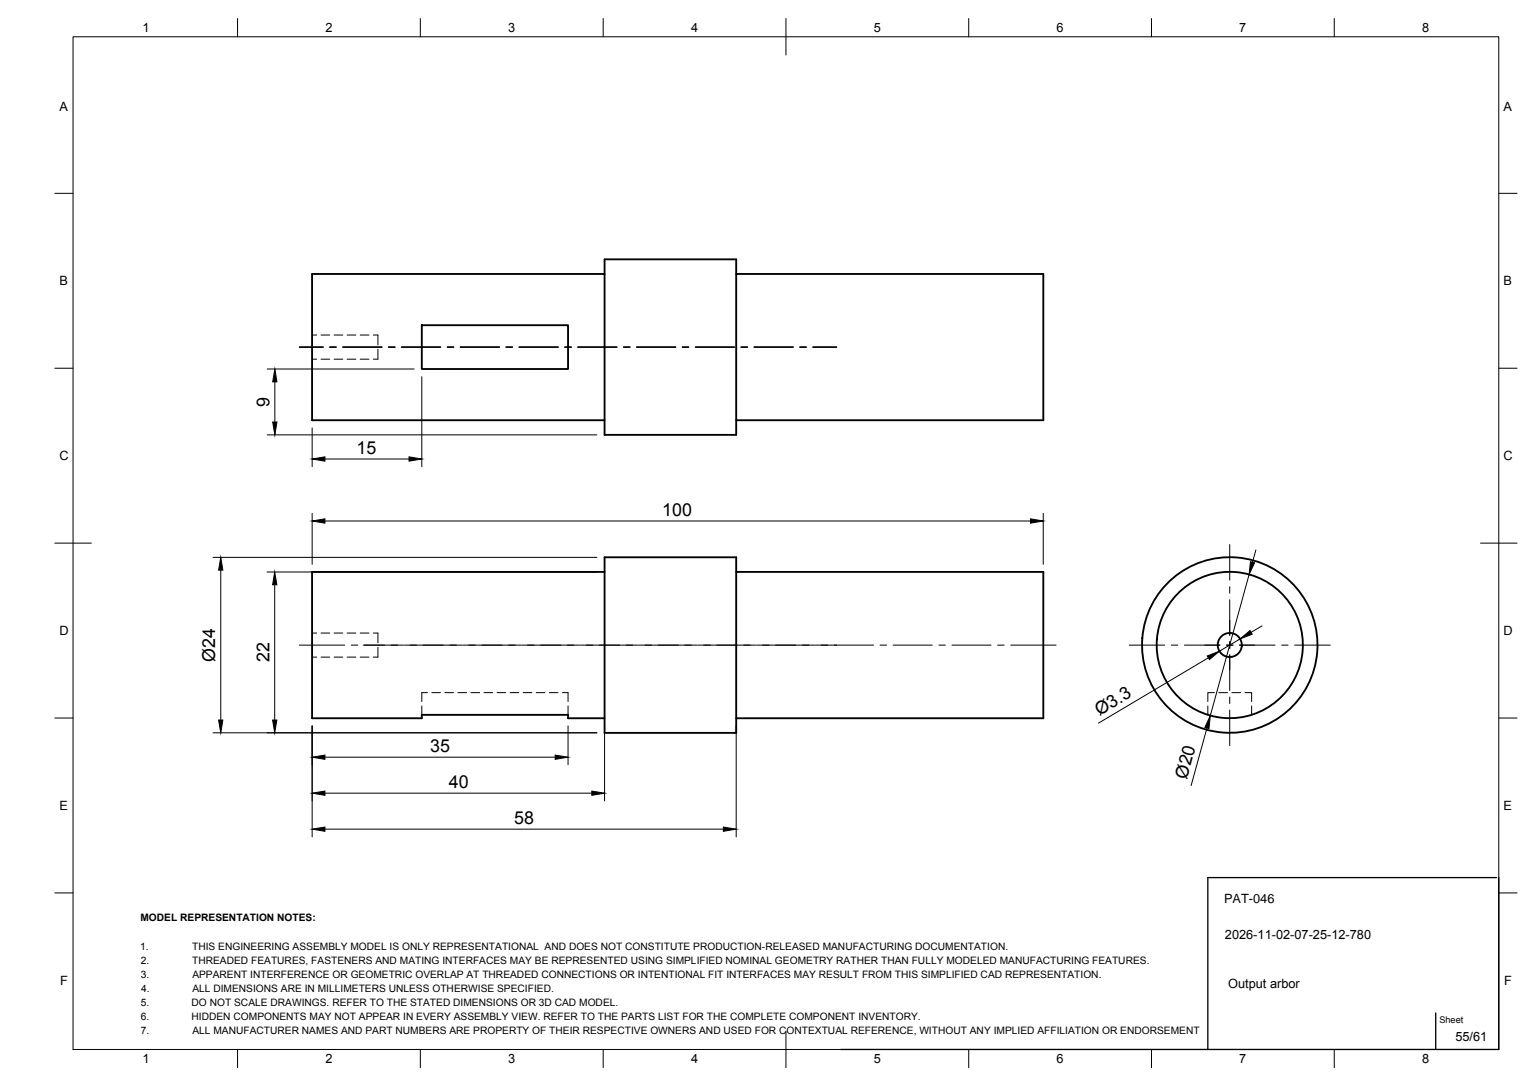
ISO-10303-21;
HEADER;
/* Generated by software containing ST-Developer
 * from STEP Tools, Inc. (www.steptools.com) 
 */

FILE_DESCRIPTION(
/* description */ ('Gear mesh backlash fixture'),
/* implementation_level */ '2;1');

FILE_NAME(
/* name */ 'Output arbor.step',
/* time_stamp */ '2026-10-28T03:26:00-07:00',
/* author */ (''),
/* organization */ (''),
/* preprocessor_version */ 'ST-DEVELOPER v20.2',
/* originating_system */ 'Autodesk Translation Framework v15.17.0.0',
/* authorisation */ '');

FILE_SCHEMA (('AUTOMOTIVE_DESIGN { 1 0 10303 214 3 1 1 }'));
ENDSEC;

DATA;
#10=MECHANICAL_DESIGN_GEOMETRIC_PRESENTATION_REPRESENTATION('',(#1072),#57900);
#957=SHAPE_REPRESENTATION_RELATIONSHIP('SRR','None',#58158,#1007);
#1007=ADVANCED_BREP_SHAPE_REPRESENTATION('',(#1135),#57891);
#1072=STYLED_ITEM('',(#58479),#1135);
#1135=MANIFOLD_SOLID_BREP('Body1',#13634);
#1311=FACE_BOUND('',#3168,.T.);
#1312=FACE_BOUND('',#3170,.T.);
#1313=FACE_BOUND('',#3174,.T.);
#1314=FACE_BOUND('',#3176,.T.);
#1604=PLANE('',#15226);
#1605=PLANE('',#15227);
#1606=PLANE('',#15228);
#1607=PLANE('',#15230);
#1608=PLANE('',#15231);
#1609=PLANE('',#15232);
#1610=PLANE('',#15234);
#1611=PLANE('',#15237);
#1612=PLANE('',#15245);
#1613=PLANE('',#15246);
#2227=FACE_OUTER_BOUND('',#3160,.T.);
#2228=FACE_OUTER_BOUND('',#3161,.T.);
#2229=FACE_OUTER_BOUND('',#3162,.T.);
#2230=FACE_OUTER_BOUND('',#3163,.T.);
#2231=FACE_OUTER_BOUND('',#3164,.T.);
#2232=FACE_OUTER_BOUND('',#3165,.T.);
#2233=FACE_OUTER_BOUND('',#3166,.T.);
#2234=FACE_OUTER_BOUND('',#3167,.T.);
#2235=FACE_OUTER_BOUND('',#3169,.T.);
#2236=FACE_OUTER_BOUND('',#3171,.T.);
#2237=FACE_OUTER_BOUND('',#3172,.T.);
#2238=FACE_OUTER_BOUND('',#3173,.T.);
#2239=FACE_OUTER_BOUND('',#3175,.T.);
#2240=FACE_OUTER_BOUND('',#3177,.T.);
#3160=EDGE_LOOP('',(#11359,#11360,#11361,#11362));
#3161=EDGE_LOOP('',(#11363));
#3162=EDGE_LOOP('',(#11364,#11365,#11366,#11367));
#3163=EDGE_LOOP('',(#11368,#11369,#11370,#11371));
#3164=EDGE_LOOP('',(#11372,#11373,#11374,#11375));
#3165=EDGE_LOOP('',(#11376,#11377,#11378,#11379));
#3166=EDGE_LOOP('',(#11380,#11381,#11382,#11383));
#3167=EDGE_LOOP('',(#11384));
#3168=EDGE_LOOP('',(#11385));
#3169=EDGE_LOOP('',(#11386));
#3170=EDGE_LOOP('',(#11387));
#3171=EDGE_LOOP('',(#11388,#11389,#11390,#11391));
#3172=EDGE_LOOP('',(#11392,#11393,#11394,#11395));
#3173=EDGE_LOOP('',(#11396,#11397,#11398,#11399));
#3174=EDGE_LOOP('',(#11400,#11401,#11402,#11403));
#3175=EDGE_LOOP('',(#11404));
#3176=EDGE_LOOP('',(#11405));
#3177=EDGE_LOOP('',(#11406));
#4051=LINE('',#33823,#4940);
#4052=LINE('',#33829,#4941);
#4053=LINE('',#33831,#4942);
#4054=LINE('',#33833,#4943);
#4055=LINE('',#33834,#4944);
#4056=LINE('',#33839,#4945);
#4057=LINE('',#33840,#4946);
#4058=LINE('',#33843,#4947);
#4059=LINE('',#33844,#4948);
#4060=LINE('',#33847,#4949);
#4061=LINE('',#33848,#4950);
#4062=LINE('',#33862,#4951);
#4063=LINE('',#33865,#4952);
#4064=LINE('',#33870,#4953);
#4940=VECTOR('',#18278,0.165);
#4941=VECTOR('',#18285,1.);
#4942=VECTOR('',#18286,1.);
#4943=VECTOR('',#18287,1.);
#4944=VECTOR('',#18288,1.);
#4945=VECTOR('',#18293,1.);
#4946=VECTOR('',#18294,1.);
#4947=VECTOR('',#18297,1.);
#4948=VECTOR('',#18298,1.);
#4949=VECTOR('',#18301,1.);
#4950=VECTOR('',#18302,1.);
#4951=VECTOR('',#18321,1.2);
#4952=VECTOR('',#18324,1.);
#4953=VECTOR('',#18331,1.);
#5661=CIRCLE('',#15224,0.165);
#5662=CIRCLE('',#15225,0.165);
#5663=CIRCLE('',#15229,1.);
#5664=CIRCLE('',#15233,1.);
#5665=CIRCLE('',#15235,1.2);
#5666=CIRCLE('',#15236,1.);
#5667=CIRCLE('',#15238,1.2);
#5668=CIRCLE('',#15239,1.);
#5669=CIRCLE('',#15242,1.);
#5670=CIRCLE('',#15244,1.);
#6618=VERTEX_POINT('',#33820);
#6619=VERTEX_POINT('',#33822);
#6620=VERTEX_POINT('',#33827);
#6621=VERTEX_POINT('',#33828);
#6622=VERTEX_POINT('',#33830);
#6623=VERTEX_POINT('',#33832);
#6624=VERTEX_POINT('',#33836);
#6625=VERTEX_POINT('',#33838);
#6626=VERTEX_POINT('',#33842);
#6627=VERTEX_POINT('',#33846);
#6628=VERTEX_POINT('',#33852);
#6629=VERTEX_POINT('',#33854);
#6630=VERTEX_POINT('',#33857);
#6631=VERTEX_POINT('',#33859);
#6632=VERTEX_POINT('',#33864);
#6633=VERTEX_POINT('',#33868);
#8266=EDGE_CURVE('',#6618,#6618,#5661,.T.);
#8267=EDGE_CURVE('',#6618,#6619,#4051,.T.);
#8268=EDGE_CURVE('',#6619,#6619,#5662,.T.);
#8269=EDGE_CURVE('',#6620,#6621,#4052,.T.);
#8270=EDGE_CURVE('',#6620,#6622,#4053,.T.);
#8271=EDGE_CURVE('',#6623,#6622,#4054,.T.);
#8272=EDGE_CURVE('',#6623,#6621,#4055,.T.);
#8273=EDGE_CURVE('',#6621,#6624,#5663,.T.);
#8274=EDGE_CURVE('',#6625,#6623,#4056,.T.);
#8275=EDGE_CURVE('',#6624,#6625,#4057,.T.);
#8276=EDGE_CURVE('',#6622,#6626,#4058,.T.);
#8277=EDGE_CURVE('',#6625,#6626,#4059,.T.);
#8278=EDGE_CURVE('',#6624,#6627,#4060,.T.);
#8279=EDGE_CURVE('',#6626,#6627,#4061,.T.);
#8280=EDGE_CURVE('',#6627,#6620,#5664,.T.);
#8281=EDGE_CURVE('',#6628,#6628,#5665,.T.);
#8282=EDGE_CURVE('',#6629,#6629,#5666,.T.);
#8283=EDGE_CURVE('',#6630,#6630,#5667,.T.);
#8284=EDGE_CURVE('',#6631,#6631,#5668,.T.);
#8285=EDGE_CURVE('',#6628,#6630,#4062,.T.);
#8286=EDGE_CURVE('',#6631,#6632,#4063,.T.);
#8287=EDGE_CURVE('',#6632,#6632,#5669,.T.);
#8288=EDGE_CURVE('',#6633,#6633,#5670,.T.);
#8289=EDGE_CURVE('',#6633,#6629,#4064,.T.);
#11359=ORIENTED_EDGE('',*,*,#8266,.F.);
#11360=ORIENTED_EDGE('',*,*,#8267,.T.);
#11361=ORIENTED_EDGE('',*,*,#8268,.F.);
#11362=ORIENTED_EDGE('',*,*,#8267,.F.);
#11363=ORIENTED_EDGE('',*,*,#8266,.T.);
#11364=ORIENTED_EDGE('',*,*,#8269,.F.);
#11365=ORIENTED_EDGE('',*,*,#8270,.T.);
#11366=ORIENTED_EDGE('',*,*,#8271,.F.);
#11367=ORIENTED_EDGE('',*,*,#8272,.T.);
#11368=ORIENTED_EDGE('',*,*,#8273,.F.);
#11369=ORIENTED_EDGE('',*,*,#8272,.F.);
#11370=ORIENTED_EDGE('',*,*,#8274,.F.);
#11371=ORIENTED_EDGE('',*,*,#8275,.F.);
#11372=ORIENTED_EDGE('',*,*,#8274,.T.);
#11373=ORIENTED_EDGE('',*,*,#8271,.T.);
#11374=ORIENTED_EDGE('',*,*,#8276,.T.);
#11375=ORIENTED_EDGE('',*,*,#8277,.F.);
#11376=ORIENTED_EDGE('',*,*,#8278,.F.);
#11377=ORIENTED_EDGE('',*,*,#8275,.T.);
#11378=ORIENTED_EDGE('',*,*,#8277,.T.);
#11379=ORIENTED_EDGE('',*,*,#8279,.T.);
#11380=ORIENTED_EDGE('',*,*,#8280,.F.);
#11381=ORIENTED_EDGE('',*,*,#8279,.F.);
#11382=ORIENTED_EDGE('',*,*,#8276,.F.);
#11383=ORIENTED_EDGE('',*,*,#8270,.F.);
#11384=ORIENTED_EDGE('',*,*,#8281,.T.);
#11385=ORIENTED_EDGE('',*,*,#8282,.F.);
#11386=ORIENTED_EDGE('',*,*,#8283,.F.);
#11387=ORIENTED_EDGE('',*,*,#8284,.F.);
#11388=ORIENTED_EDGE('',*,*,#8281,.F.);
#11389=ORIENTED_EDGE('',*,*,#8285,.T.);
#11390=ORIENTED_EDGE('',*,*,#8283,.T.);
#11391=ORIENTED_EDGE('',*,*,#8285,.F.);
#11392=ORIENTED_EDGE('',*,*,#8284,.T.);
#11393=ORIENTED_EDGE('',*,*,#8286,.T.);
#11394=ORIENTED_EDGE('',*,*,#8287,.T.);
#11395=ORIENTED_EDGE('',*,*,#8286,.F.);
#11396=ORIENTED_EDGE('',*,*,#8288,.F.);
#11397=ORIENTED_EDGE('',*,*,#8289,.T.);
#11398=ORIENTED_EDGE('',*,*,#8282,.T.);
#11399=ORIENTED_EDGE('',*,*,#8289,.F.);
#11400=ORIENTED_EDGE('',*,*,#8278,.T.);
#11401=ORIENTED_EDGE('',*,*,#8280,.T.);
#11402=ORIENTED_EDGE('',*,*,#8269,.T.);
#11403=ORIENTED_EDGE('',*,*,#8273,.T.);
#11404=ORIENTED_EDGE('',*,*,#8288,.T.);
#11405=ORIENTED_EDGE('',*,*,#8268,.T.);
#11406=ORIENTED_EDGE('',*,*,#8287,.F.);
#12753=CYLINDRICAL_SURFACE('',#15223,0.165);
#12754=CYLINDRICAL_SURFACE('',#15240,1.2);
#12755=CYLINDRICAL_SURFACE('',#15241,1.);
#12756=CYLINDRICAL_SURFACE('',#15243,1.);
#13344=ADVANCED_FACE('',(#2227),#12753,.F.);
#13345=ADVANCED_FACE('',(#2228),#1604,.T.);
#13346=ADVANCED_FACE('',(#2229),#1605,.F.);
#13347=ADVANCED_FACE('',(#2230),#1606,.T.);
#13348=ADVANCED_FACE('',(#2231),#1607,.F.);
#13349=ADVANCED_FACE('',(#2232),#1608,.F.);
#13350=ADVANCED_FACE('',(#2233),#1609,.F.);
#13351=ADVANCED_FACE('',(#2234,#1311),#1610,.T.);
#13352=ADVANCED_FACE('',(#2235,#1312),#1611,.F.);
#13353=ADVANCED_FACE('',(#2236),#12754,.T.);
#13354=ADVANCED_FACE('',(#2237),#12755,.T.);
#13355=ADVANCED_FACE('',(#2238,#1313),#12756,.T.);
#13356=ADVANCED_FACE('',(#2239,#1314),#1612,.T.);
#13357=ADVANCED_FACE('',(#2240),#1613,.F.);
#13634=CLOSED_SHELL('',(#13344,#13345,#13346,#13347,#13348,#13349,#13350,
#13351,#13352,#13353,#13354,#13355,#13356,#13357));
#15222=AXIS2_PLACEMENT_3D('',#33818,#18272,#18273);
#15223=AXIS2_PLACEMENT_3D('',#33819,#18274,#18275);
#15224=AXIS2_PLACEMENT_3D('',#33821,#18276,#18277);
#15225=AXIS2_PLACEMENT_3D('',#33824,#18279,#18280);
#15226=AXIS2_PLACEMENT_3D('',#33825,#18281,#18282);
#15227=AXIS2_PLACEMENT_3D('',#33826,#18283,#18284);
#15228=AXIS2_PLACEMENT_3D('',#33835,#18289,#18290);
#15229=AXIS2_PLACEMENT_3D('',#33837,#18291,#18292);
#15230=AXIS2_PLACEMENT_3D('',#33841,#18295,#18296);
#15231=AXIS2_PLACEMENT_3D('',#33845,#18299,#18300);
#15232=AXIS2_PLACEMENT_3D('',#33849,#18303,#18304);
#15233=AXIS2_PLACEMENT_3D('',#33850,#18305,#18306);
#15234=AXIS2_PLACEMENT_3D('',#33851,#18307,#18308);
#15235=AXIS2_PLACEMENT_3D('',#33853,#18309,#18310);
#15236=AXIS2_PLACEMENT_3D('',#33855,#18311,#18312);
#15237=AXIS2_PLACEMENT_3D('',#33856,#18313,#18314);
#15238=AXIS2_PLACEMENT_3D('',#33858,#18315,#18316);
#15239=AXIS2_PLACEMENT_3D('',#33860,#18317,#18318);
#15240=AXIS2_PLACEMENT_3D('',#33861,#18319,#18320);
#15241=AXIS2_PLACEMENT_3D('',#33863,#18322,#18323);
#15242=AXIS2_PLACEMENT_3D('',#33866,#18325,#18326);
#15243=AXIS2_PLACEMENT_3D('',#33867,#18327,#18328);
#15244=AXIS2_PLACEMENT_3D('',#33869,#18329,#18330);
#15245=AXIS2_PLACEMENT_3D('',#33871,#18332,#18333);
#15246=AXIS2_PLACEMENT_3D('',#33872,#18334,#18335);
#18272=DIRECTION('axis',(0.,0.,1.));
#18273=DIRECTION('refdir',(1.,0.,0.));
#18274=DIRECTION('center_axis',(0.,0.,1.));
#18275=DIRECTION('ref_axis',(1.,0.,0.));
#18276=DIRECTION('center_axis',(0.,0.,1.));
#18277=DIRECTION('ref_axis',(1.,0.,0.));
#18278=DIRECTION('',(0.,0.,1.));
#18279=DIRECTION('center_axis',(0.,0.,-1.));
#18280=DIRECTION('ref_axis',(1.,0.,0.));
#18281=DIRECTION('center_axis',(0.,0.,1.));
#18282=DIRECTION('ref_axis',(1.,0.,0.));
#18283=DIRECTION('center_axis',(-0.996917333733128,-0.0784590957278475,
0.));
#18284=DIRECTION('ref_axis',(0.0784590957278475,-0.996917333733128,0.));
#18285=DIRECTION('',(0.,0.,-1.));
#18286=DIRECTION('',(0.0784590957278475,-0.996917333733128,0.));
#18287=DIRECTION('',(0.,0.,1.));
#18288=DIRECTION('',(-0.0784590957278475,0.996917333733128,0.));
#18289=DIRECTION('center_axis',(0.,0.,1.));
#18290=DIRECTION('ref_axis',(1.,0.,0.));
#18291=DIRECTION('center_axis',(0.,0.,-1.));
#18292=DIRECTION('ref_axis',(1.,0.,0.));
#18293=DIRECTION('',(-0.996917333733128,-0.0784590957278448,0.));
#18294=DIRECTION('',(0.0784590957278475,-0.996917333733128,0.));
#18295=DIRECTION('center_axis',(0.0784590957278448,-0.996917333733128,0.));
#18296=DIRECTION('ref_axis',(0.996917333733128,0.0784590957278448,0.));
#18297=DIRECTION('',(0.996917333733128,0.0784590957278448,0.));
#18298=DIRECTION('',(0.,0.,1.));
#18299=DIRECTION('center_axis',(0.996917333733128,0.0784590957278475,0.));
#18300=DIRECTION('ref_axis',(-0.0784590957278475,0.996917333733128,0.));
#18301=DIRECTION('',(0.,0.,1.));
#18302=DIRECTION('',(-0.0784590957278475,0.996917333733128,0.));
#18303=DIRECTION('center_axis',(0.,0.,1.));
#18304=DIRECTION('ref_axis',(1.,0.,0.));
#18305=DIRECTION('center_axis',(0.,0.,1.));
#18306=DIRECTION('ref_axis',(1.,0.,0.));
#18307=DIRECTION('center_axis',(0.,0.,1.));
#18308=DIRECTION('ref_axis',(1.,0.,0.));
#18309=DIRECTION('center_axis',(0.,0.,1.));
#18310=DIRECTION('ref_axis',(1.,0.,0.));
#18311=DIRECTION('center_axis',(0.,0.,1.));
#18312=DIRECTION('ref_axis',(1.,0.,0.));
#18313=DIRECTION('center_axis',(0.,0.,1.));
#18314=DIRECTION('ref_axis',(1.,0.,0.));
#18315=DIRECTION('center_axis',(0.,0.,1.));
#18316=DIRECTION('ref_axis',(1.,0.,0.));
#18317=DIRECTION('center_axis',(0.,0.,-1.));
#18318=DIRECTION('ref_axis',(1.,0.,0.));
#18319=DIRECTION('center_axis',(0.,0.,1.));
#18320=DIRECTION('ref_axis',(1.,0.,0.));
#18321=DIRECTION('',(0.,0.,-1.));
#18322=DIRECTION('center_axis',(0.,0.,1.));
#18323=DIRECTION('ref_axis',(1.,0.,0.));
#18324=DIRECTION('',(0.,0.,-1.));
#18325=DIRECTION('center_axis',(0.,0.,1.));
#18326=DIRECTION('ref_axis',(1.,0.,0.));
#18327=DIRECTION('center_axis',(0.,0.,1.));
#18328=DIRECTION('ref_axis',(1.,0.,0.));
#18329=DIRECTION('center_axis',(0.,0.,1.));
#18330=DIRECTION('ref_axis',(1.,0.,0.));
#18331=DIRECTION('',(0.,0.,-1.));
#18332=DIRECTION('center_axis',(0.,0.,1.));
#18333=DIRECTION('ref_axis',(1.,0.,0.));
#18334=DIRECTION('center_axis',(0.,0.,1.));
#18335=DIRECTION('ref_axis',(1.,0.,0.));
#33818=CARTESIAN_POINT('',(0.,0.,0.));
#33819=CARTESIAN_POINT('Origin',(6.,0.,14.1));
#33820=CARTESIAN_POINT('',(5.835,-2.02066721859313E-17,14.1));
#33821=CARTESIAN_POINT('Origin',(6.,0.,14.1));
#33822=CARTESIAN_POINT('',(5.835,2.02066721859313E-17,15.));
#33823=CARTESIAN_POINT('',(5.835,-2.02066721859313E-17,14.1));
#33824=CARTESIAN_POINT('Origin',(6.,0.,15.));
#33825=CARTESIAN_POINT('Origin',(6.,0.,14.1));
#33826=CARTESIAN_POINT('Origin',(5.61461979457943,1.07307133838809,11.5));
#33827=CARTESIAN_POINT('',(5.62607959275755,0.927460796501737,13.5));
#33828=CARTESIAN_POINT('',(5.62607959275755,0.927460796501737,11.5));
#33829=CARTESIAN_POINT('',(5.62607959275755,0.927460796501737,5.));
#33830=CARTESIAN_POINT('',(5.64992638765696,0.62445853820818,13.5));
#33831=CARTESIAN_POINT('',(5.64992638765696,0.62445853820818,13.5));
#33832=CARTESIAN_POINT('',(5.64992638765696,0.62445853820818,11.5));
#33833=CARTESIAN_POINT('',(5.64992638765696,0.62445853820818,11.5));
#33834=CARTESIAN_POINT('',(5.64992638765696,0.62445853820818,11.5));
#33835=CARTESIAN_POINT('Origin',(5.93134829123814,0.872302667016487,11.5));
#33836=CARTESIAN_POINT('',(6.22422999299742,0.974536253938444,11.5));
#33837=CARTESIAN_POINT('Origin',(6.,0.,11.5));
#33838=CARTESIAN_POINT('',(6.24807678789684,0.671533995644887,11.5));
#33839=CARTESIAN_POINT('',(6.24807678789684,0.671533995644887,11.5));
#33840=CARTESIAN_POINT('',(6.21277019481931,1.12014679582479,11.5));
#33841=CARTESIAN_POINT('Origin',(5.64992638765696,0.62445853820818,11.5));
#33842=CARTESIAN_POINT('',(6.24807678789684,0.671533995644887,13.5));
#33843=CARTESIAN_POINT('',(6.24807678789684,0.671533995644887,13.5));
#33844=CARTESIAN_POINT('',(6.24807678789684,0.671533995644887,11.5));
#33845=CARTESIAN_POINT('Origin',(6.24807678789684,0.671533995644887,11.5));
#33846=CARTESIAN_POINT('',(6.22422999299742,0.974536253938444,13.5));
#33847=CARTESIAN_POINT('',(6.22422999299742,0.974536253938444,5.));
#33848=CARTESIAN_POINT('',(6.21277019481931,1.12014679582479,13.5));
#33849=CARTESIAN_POINT('Origin',(5.93134829123814,0.872302667016487,13.5));
#33850=CARTESIAN_POINT('Origin',(6.,0.,13.5));
#33851=CARTESIAN_POINT('Origin',(6.,0.,11.));
#33852=CARTESIAN_POINT('',(4.8,-1.46957615897682E-16,11.));
#33853=CARTESIAN_POINT('Origin',(6.,0.,11.));
#33854=CARTESIAN_POINT('',(5.,-1.22464679914735E-16,11.));
#33855=CARTESIAN_POINT('Origin',(6.,0.,11.));
#33856=CARTESIAN_POINT('Origin',(6.,0.,9.2));
#33857=CARTESIAN_POINT('',(4.8,-1.46957615897682E-16,9.2));
#33858=CARTESIAN_POINT('Origin',(6.,0.,9.2));
#33859=CARTESIAN_POINT('',(5.,1.22464679914735E-16,9.2));
#33860=CARTESIAN_POINT('Origin',(6.,0.,9.2));
#33861=CARTESIAN_POINT('Origin',(6.,0.,9.2));
#33862=CARTESIAN_POINT('',(4.8,-1.46957615897682E-16,9.2));
#33863=CARTESIAN_POINT('Origin',(6.,0.,5.));
#33864=CARTESIAN_POINT('',(5.,-1.22464679914735E-16,5.));
#33865=CARTESIAN_POINT('',(5.,-1.22464679914735E-16,5.));
#33866=CARTESIAN_POINT('Origin',(6.,0.,5.));
#33867=CARTESIAN_POINT('Origin',(6.,0.,5.));
#33868=CARTESIAN_POINT('',(5.,-1.22464679914735E-16,15.));
#33869=CARTESIAN_POINT('Origin',(6.,0.,15.));
#33870=CARTESIAN_POINT('',(5.,-1.22464679914735E-16,5.));
#33871=CARTESIAN_POINT('Origin',(6.,0.,15.));
#33872=CARTESIAN_POINT('Origin',(6.,0.,5.));
#57832=UNCERTAINTY_MEASURE_WITH_UNIT(LENGTH_MEASURE(0.001),#57901,
'DISTANCE_ACCURACY_VALUE',
'Maximum model space distance between geometric entities at asserted c
onnectivities');
#57841=UNCERTAINTY_MEASURE_WITH_UNIT(LENGTH_MEASURE(0.001),#57901,
'DISTANCE_ACCURACY_VALUE',
'Maximum model space distance between geometric entities at asserted c
onnectivities');
#57891=(
GEOMETRIC_REPRESENTATION_CONTEXT(3)
GLOBAL_UNCERTAINTY_ASSIGNED_CONTEXT((#57832))
GLOBAL_UNIT_ASSIGNED_CONTEXT((#57901,#57903,#57904))
REPRESENTATION_CONTEXT('','3D')
);
#57900=(
GEOMETRIC_REPRESENTATION_CONTEXT(3)
GLOBAL_UNCERTAINTY_ASSIGNED_CONTEXT((#57841))
GLOBAL_UNIT_ASSIGNED_CONTEXT((#57901,#57903,#57904))
REPRESENTATION_CONTEXT('','3D')
);
#57901=(
LENGTH_UNIT()
NAMED_UNIT(*)
SI_UNIT(.CENTI.,.METRE.)
);
#57903=(
NAMED_UNIT(*)
PLANE_ANGLE_UNIT()
SI_UNIT($,.RADIAN.)
);
#57904=(
NAMED_UNIT(*)
SI_UNIT($,.STERADIAN.)
SOLID_ANGLE_UNIT()
);
#57954=SHAPE_DEFINITION_REPRESENTATION(#58025,#58158);
#58025=PRODUCT_DEFINITION_SHAPE('',$,#58217);
#58158=SHAPE_REPRESENTATION('',(#15222),#57891);
#58167=PRODUCT_DEFINITION_CONTEXT('part definition',#58343,'design');
#58217=PRODUCT_DEFINITION('Output arbor','Output arbor',#58275,#58167);
#58275=PRODUCT_DEFINITION_FORMATION('',$,#58394);
#58343=APPLICATION_CONTEXT(
'Core Data for Automotive Mechanical Design Process');
#58344=PRODUCT_CONTEXT('part definition',#58343,'mechanical');
#58394=PRODUCT('Output arbor','Output arbor','Output arbor',(#58344));
#58473=COLOUR_RGB('Off White',0.89,0.88,0.83);
#58474=FILL_AREA_STYLE_COLOUR('',#58473);
#58475=FILL_AREA_STYLE('',(#58474));
#58476=SURFACE_STYLE_FILL_AREA(#58475);
#58477=SURFACE_SIDE_STYLE('',(#58476));
#58478=SURFACE_STYLE_USAGE(.BOTH.,#58477);
#58479=PRESENTATION_STYLE_ASSIGNMENT((#58478));
ENDSEC;
END-ISO-10303-21;
